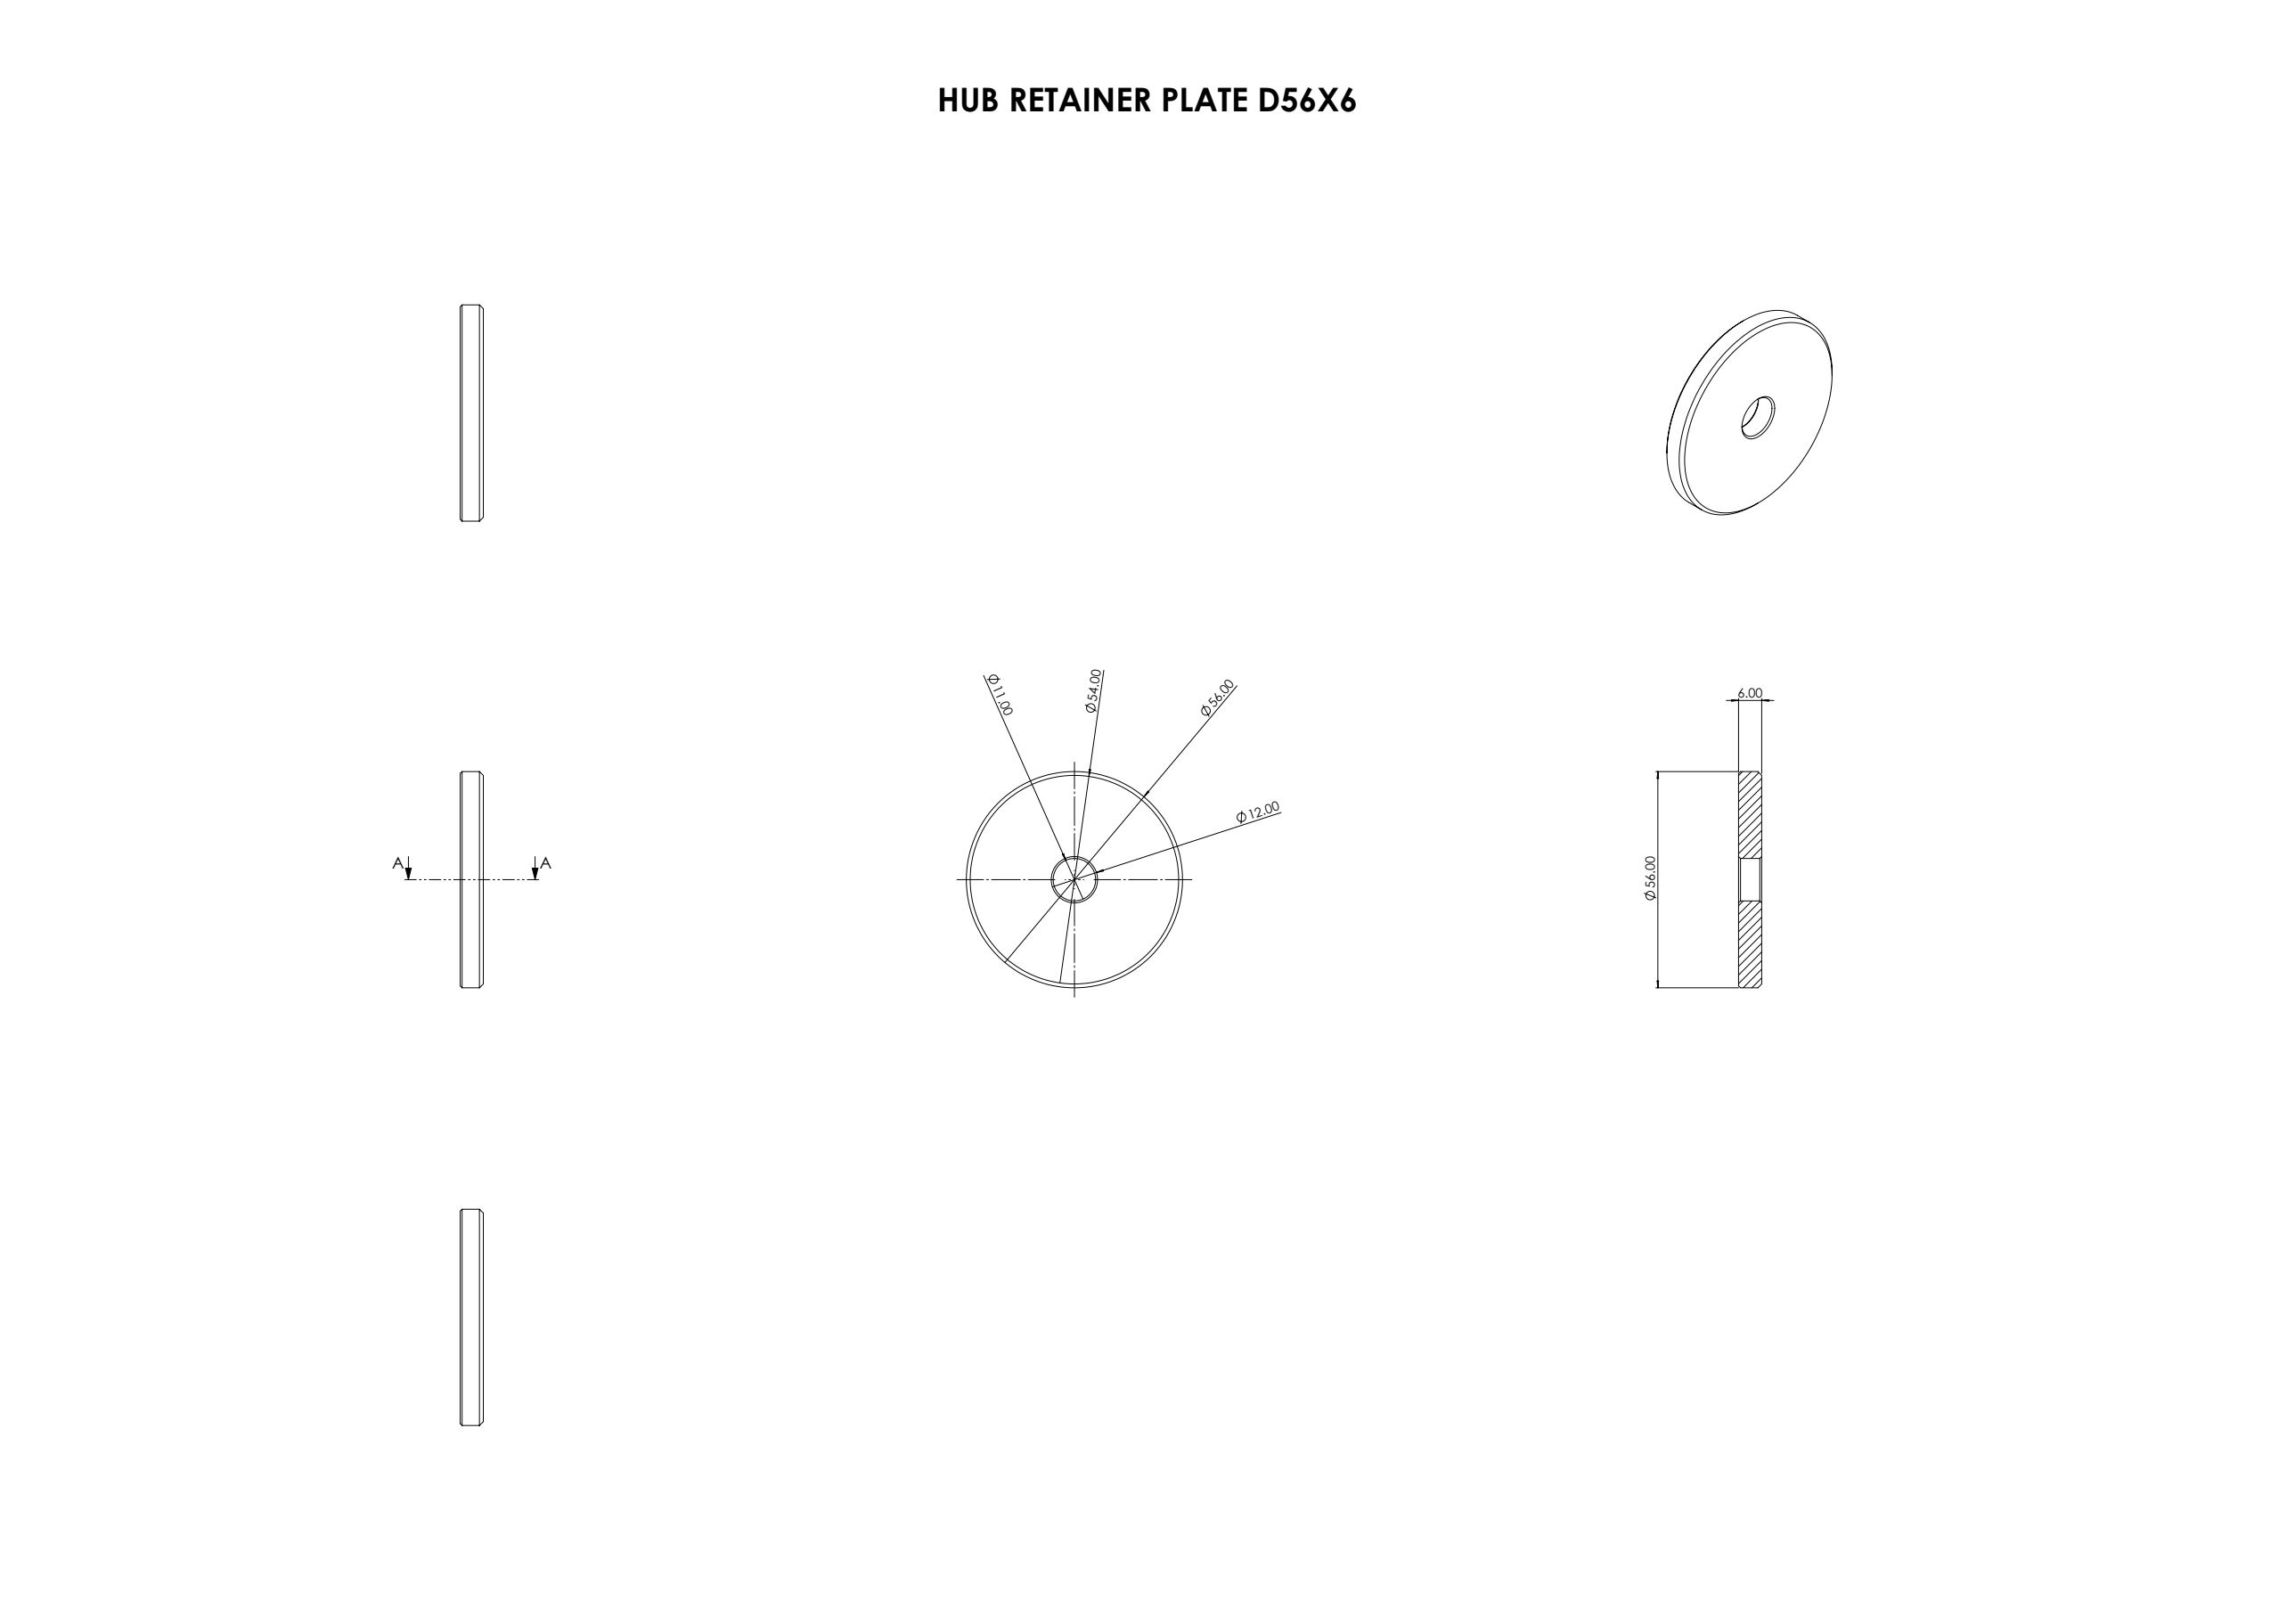
ISO-10303-21;
HEADER;
/* Generated by software containing ST-Developer
 * from STEP Tools, Inc. (www.steptools.com) 
 */

FILE_DESCRIPTION(
/* description */ (''),
/* implementation_level */ '2;1');

FILE_NAME(
/* name */ '05_Hub_Retainer_Plate_D56x6.step',
/* time_stamp */ '2026-10-11T08:27:52-07:00',
/* author */ (''),
/* organization */ (''),
/* preprocessor_version */ 'ST-DEVELOPER v20.2',
/* originating_system */ 'Autodesk Translation Framework v15.15.0.0',
/* authorisation */ '');

FILE_SCHEMA (('AUTOMOTIVE_DESIGN { 1 0 10303 214 3 1 1 }'));
ENDSEC;

DATA;
#10=MECHANICAL_DESIGN_GEOMETRIC_PRESENTATION_REPRESENTATION('',(#923),#94301);
#895=SHAPE_REPRESENTATION_RELATIONSHIP('SRR','None',#94375,#909);
#909=ADVANCED_BREP_SHAPE_REPRESENTATION('',(#937),#94291);
#923=STYLED_ITEM('',(#94574),#937);
#937=MANIFOLD_SOLID_BREP('Body1',#51022);
#1028=FACE_BOUND('',#18160,.T.);
#1029=FACE_BOUND('',#18165,.T.);
#1155=CYLINDRICAL_SURFACE('',#54475,5.5);
#1156=CYLINDRICAL_SURFACE('',#54484,28.);
#5973=LINE('',#84055,#10501);
#5974=LINE('',#84059,#10502);
#5975=LINE('',#84067,#10503);
#5976=LINE('',#84071,#10504);
#5977=LINE('',#84075,#10505);
#5978=LINE('',#84080,#10506);
#10501=VECTOR('',#65761,5.5);
#10502=VECTOR('',#65766,5.75);
#10503=VECTOR('',#65777,27.75);
#10504=VECTOR('',#65782,28.);
#10505=VECTOR('',#65787,27.5);
#10506=VECTOR('',#65794,5.75);
#12901=PLANE('',#54480);
#12902=PLANE('',#54488);
#15406=FACE_OUTER_BOUND('',#18157,.T.);
#15407=FACE_OUTER_BOUND('',#18158,.T.);
#15408=FACE_OUTER_BOUND('',#18159,.T.);
#15409=FACE_OUTER_BOUND('',#18161,.T.);
#15410=FACE_OUTER_BOUND('',#18162,.T.);
#15411=FACE_OUTER_BOUND('',#18163,.T.);
#15412=FACE_OUTER_BOUND('',#18164,.T.);
#15413=FACE_OUTER_BOUND('',#18166,.T.);
#18157=EDGE_LOOP('',(#45475,#45476,#45477,#45478));
#18158=EDGE_LOOP('',(#45479,#45480,#45481,#45482));
#18159=EDGE_LOOP('',(#45483));
#18160=EDGE_LOOP('',(#45484));
#18161=EDGE_LOOP('',(#45485,#45486,#45487,#45488));
#18162=EDGE_LOOP('',(#45489,#45490,#45491,#45492));
#18163=EDGE_LOOP('',(#45493,#45494,#45495,#45496));
#18164=EDGE_LOOP('',(#45497));
#18165=EDGE_LOOP('',(#45498));
#18166=EDGE_LOOP('',(#45499,#45500,#45501,#45502));
#20001=CIRCLE('',#54476,5.5);
#20002=CIRCLE('',#54477,5.5);
#20003=CIRCLE('',#54479,6.);
#20004=CIRCLE('',#54481,27.5);
#20005=CIRCLE('',#54483,28.);
#20006=CIRCLE('',#54485,28.);
#20007=CIRCLE('',#54487,27.);
#20008=CIRCLE('',#54489,6.);
#24498=VERTEX_POINT('',#84052);
#24499=VERTEX_POINT('',#84054);
#24500=VERTEX_POINT('',#84058);
#24501=VERTEX_POINT('',#84062);
#24502=VERTEX_POINT('',#84065);
#24503=VERTEX_POINT('',#84069);
#24504=VERTEX_POINT('',#84073);
#24505=VERTEX_POINT('',#84077);
#31599=EDGE_CURVE('',#24498,#24498,#20001,.T.);
#31600=EDGE_CURVE('',#24498,#24499,#5973,.T.);
#31601=EDGE_CURVE('',#24499,#24499,#20002,.T.);
#31602=EDGE_CURVE('',#24499,#24500,#5974,.T.);
#31603=EDGE_CURVE('',#24500,#24500,#20003,.T.);
#31604=EDGE_CURVE('',#24501,#24501,#20004,.T.);
#31605=EDGE_CURVE('',#24502,#24502,#20005,.T.);
#31606=EDGE_CURVE('',#24502,#24501,#5975,.T.);
#31607=EDGE_CURVE('',#24503,#24503,#20006,.T.);
#31608=EDGE_CURVE('',#24503,#24502,#5976,.T.);
#31609=EDGE_CURVE('',#24504,#24504,#20007,.T.);
#31610=EDGE_CURVE('',#24504,#24503,#5977,.T.);
#31611=EDGE_CURVE('',#24505,#24505,#20008,.T.);
#31612=EDGE_CURVE('',#24505,#24498,#5978,.T.);
#45475=ORIENTED_EDGE('',*,*,#31599,.T.);
#45476=ORIENTED_EDGE('',*,*,#31600,.T.);
#45477=ORIENTED_EDGE('',*,*,#31601,.F.);
#45478=ORIENTED_EDGE('',*,*,#31600,.F.);
#45479=ORIENTED_EDGE('',*,*,#31601,.T.);
#45480=ORIENTED_EDGE('',*,*,#31602,.T.);
#45481=ORIENTED_EDGE('',*,*,#31603,.F.);
#45482=ORIENTED_EDGE('',*,*,#31602,.F.);
#45483=ORIENTED_EDGE('',*,*,#31604,.F.);
#45484=ORIENTED_EDGE('',*,*,#31603,.T.);
#45485=ORIENTED_EDGE('',*,*,#31605,.F.);
#45486=ORIENTED_EDGE('',*,*,#31606,.T.);
#45487=ORIENTED_EDGE('',*,*,#31604,.T.);
#45488=ORIENTED_EDGE('',*,*,#31606,.F.);
#45489=ORIENTED_EDGE('',*,*,#31607,.F.);
#45490=ORIENTED_EDGE('',*,*,#31608,.T.);
#45491=ORIENTED_EDGE('',*,*,#31605,.T.);
#45492=ORIENTED_EDGE('',*,*,#31608,.F.);
#45493=ORIENTED_EDGE('',*,*,#31609,.F.);
#45494=ORIENTED_EDGE('',*,*,#31610,.T.);
#45495=ORIENTED_EDGE('',*,*,#31607,.T.);
#45496=ORIENTED_EDGE('',*,*,#31610,.F.);
#45497=ORIENTED_EDGE('',*,*,#31609,.T.);
#45498=ORIENTED_EDGE('',*,*,#31611,.F.);
#45499=ORIENTED_EDGE('',*,*,#31611,.T.);
#45500=ORIENTED_EDGE('',*,*,#31612,.T.);
#45501=ORIENTED_EDGE('',*,*,#31599,.F.);
#45502=ORIENTED_EDGE('',*,*,#31612,.F.);
#48302=CONICAL_SURFACE('',#54478,5.75,0.785398163397448);
#48303=CONICAL_SURFACE('',#54482,27.75,0.785398163397447);
#48304=CONICAL_SURFACE('',#54486,27.5,0.785398163397447);
#48305=CONICAL_SURFACE('',#54490,5.75,0.785398163397448);
#50493=ADVANCED_FACE('',(#15406),#1155,.F.);
#50494=ADVANCED_FACE('',(#15407),#48302,.F.);
#50495=ADVANCED_FACE('',(#15408,#1028),#12901,.T.);
#50496=ADVANCED_FACE('',(#15409),#48303,.T.);
#50497=ADVANCED_FACE('',(#15410),#1156,.T.);
#50498=ADVANCED_FACE('',(#15411),#48304,.T.);
#50499=ADVANCED_FACE('',(#15412,#1029),#12902,.T.);
#50500=ADVANCED_FACE('',(#15413),#48305,.F.);
#51022=CLOSED_SHELL('',(#50493,#50494,#50495,#50496,#50497,#50498,#50499,
#50500));
#54474=AXIS2_PLACEMENT_3D('',#84050,#65755,#65756);
#54475=AXIS2_PLACEMENT_3D('',#84051,#65757,#65758);
#54476=AXIS2_PLACEMENT_3D('',#84053,#65759,#65760);
#54477=AXIS2_PLACEMENT_3D('',#84056,#65762,#65763);
#54478=AXIS2_PLACEMENT_3D('',#84057,#65764,#65765);
#54479=AXIS2_PLACEMENT_3D('',#84060,#65767,#65768);
#54480=AXIS2_PLACEMENT_3D('',#84061,#65769,#65770);
#54481=AXIS2_PLACEMENT_3D('',#84063,#65771,#65772);
#54482=AXIS2_PLACEMENT_3D('',#84064,#65773,#65774);
#54483=AXIS2_PLACEMENT_3D('',#84066,#65775,#65776);
#54484=AXIS2_PLACEMENT_3D('',#84068,#65778,#65779);
#54485=AXIS2_PLACEMENT_3D('',#84070,#65780,#65781);
#54486=AXIS2_PLACEMENT_3D('',#84072,#65783,#65784);
#54487=AXIS2_PLACEMENT_3D('',#84074,#65785,#65786);
#54488=AXIS2_PLACEMENT_3D('',#84076,#65788,#65789);
#54489=AXIS2_PLACEMENT_3D('',#84078,#65790,#65791);
#54490=AXIS2_PLACEMENT_3D('',#84079,#65792,#65793);
#65755=DIRECTION('axis',(0.,0.,1.));
#65756=DIRECTION('refdir',(1.,0.,0.));
#65757=DIRECTION('center_axis',(1.,0.,0.));
#65758=DIRECTION('ref_axis',(0.,1.,0.));
#65759=DIRECTION('center_axis',(1.,0.,0.));
#65760=DIRECTION('ref_axis',(0.,0.,-1.));
#65761=DIRECTION('',(-1.,0.,0.));
#65762=DIRECTION('center_axis',(1.,0.,0.));
#65763=DIRECTION('ref_axis',(0.,0.,-1.));
#65764=DIRECTION('center_axis',(-1.,0.,0.));
#65765=DIRECTION('ref_axis',(0.,1.,0.));
#65766=DIRECTION('',(-0.707106781186548,-0.707106781186547,-8.65956056235493E-17));
#65767=DIRECTION('center_axis',(1.,0.,0.));
#65768=DIRECTION('ref_axis',(0.,0.,-1.));
#65769=DIRECTION('center_axis',(-1.,0.,0.));
#65770=DIRECTION('ref_axis',(0.,0.,1.));
#65771=DIRECTION('center_axis',(1.,0.,0.));
#65772=DIRECTION('ref_axis',(0.,0.,-1.));
#65773=DIRECTION('center_axis',(1.,0.,0.));
#65774=DIRECTION('ref_axis',(0.,1.,0.));
#65775=DIRECTION('center_axis',(1.,0.,0.));
#65776=DIRECTION('ref_axis',(0.,0.,-1.));
#65777=DIRECTION('',(-0.707106781186549,0.707106781186546,8.65956056235492E-17));
#65778=DIRECTION('center_axis',(1.,0.,0.));
#65779=DIRECTION('ref_axis',(0.,1.,0.));
#65780=DIRECTION('center_axis',(1.,0.,0.));
#65781=DIRECTION('ref_axis',(0.,0.,-1.));
#65782=DIRECTION('',(-1.,0.,0.));
#65783=DIRECTION('center_axis',(-1.,0.,0.));
#65784=DIRECTION('ref_axis',(0.,1.,0.));
#65785=DIRECTION('center_axis',(1.,0.,0.));
#65786=DIRECTION('ref_axis',(0.,0.,-1.));
#65787=DIRECTION('',(-0.707106781186549,-0.707106781186546,-8.65956056235492E-17));
#65788=DIRECTION('center_axis',(1.,0.,0.));
#65789=DIRECTION('ref_axis',(0.,0.,-1.));
#65790=DIRECTION('center_axis',(1.,0.,0.));
#65791=DIRECTION('ref_axis',(0.,0.,-1.));
#65792=DIRECTION('center_axis',(1.,0.,0.));
#65793=DIRECTION('ref_axis',(0.,1.,0.));
#65794=DIRECTION('',(-0.707106781186548,0.707106781186548,8.65956056235493E-17));
#84050=CARTESIAN_POINT('',(0.,0.,0.));
#84051=CARTESIAN_POINT('Origin',(3.,0.,0.));
#84052=CARTESIAN_POINT('',(5.5,-5.5,-6.73555739531044E-16));
#84053=CARTESIAN_POINT('Origin',(5.5,0.,0.));
#84054=CARTESIAN_POINT('',(0.5,-5.5,-6.73555739531044E-16));
#84055=CARTESIAN_POINT('',(3.,-5.5,-6.73555739531044E-16));
#84056=CARTESIAN_POINT('Origin',(0.5,0.,0.));
#84057=CARTESIAN_POINT('Origin',(0.25,0.,0.));
#84058=CARTESIAN_POINT('',(-2.42861286636753E-16,-6.,-7.34788079488412E-16));
#84059=CARTESIAN_POINT('',(0.25,-5.75,-7.04171909509728E-16));
#84060=CARTESIAN_POINT('Origin',(0.,0.,0.));
#84061=CARTESIAN_POINT('Origin',(0.,27.5,0.));
#84062=CARTESIAN_POINT('',(-7.63278329429795E-16,-27.5,-3.36777869765522E-15));
#84063=CARTESIAN_POINT('Origin',(0.,0.,0.));
#84064=CARTESIAN_POINT('Origin',(0.25,0.,0.));
#84065=CARTESIAN_POINT('',(0.500000000000002,-28.,-3.42901103761259E-15));
#84066=CARTESIAN_POINT('Origin',(0.5,0.,0.));
#84067=CARTESIAN_POINT('',(0.25,-27.75,-3.39839486763391E-15));
#84068=CARTESIAN_POINT('Origin',(2.75,0.,0.));
#84069=CARTESIAN_POINT('',(5.,-28.,-3.42901103761259E-15));
#84070=CARTESIAN_POINT('Origin',(5.,0.,0.));
#84071=CARTESIAN_POINT('',(2.75,-28.,-3.42901103761259E-15));
#84072=CARTESIAN_POINT('Origin',(5.5,0.,0.));
#84073=CARTESIAN_POINT('',(6.,-27.,-3.30654635769785E-15));
#84074=CARTESIAN_POINT('Origin',(6.,0.,0.));
#84075=CARTESIAN_POINT('',(5.5,-27.5,-3.36777869765522E-15));
#84076=CARTESIAN_POINT('Origin',(6.,6.,0.));
#84077=CARTESIAN_POINT('',(6.,-6.,-7.34788079488412E-16));
#84078=CARTESIAN_POINT('Origin',(6.,0.,0.));
#84079=CARTESIAN_POINT('Origin',(5.75,0.,0.));
#84080=CARTESIAN_POINT('',(5.75,-5.75,-7.04171909509728E-16));
#94275=UNCERTAINTY_MEASURE_WITH_UNIT(LENGTH_MEASURE(0.01),#94302,
'DISTANCE_ACCURACY_VALUE',
'Maximum model space distance between geometric entities at asserted c
onnectivities');
#94285=UNCERTAINTY_MEASURE_WITH_UNIT(LENGTH_MEASURE(0.01),#94302,
'DISTANCE_ACCURACY_VALUE',
'Maximum model space distance between geometric entities at asserted c
onnectivities');
#94291=(
GEOMETRIC_REPRESENTATION_CONTEXT(3)
GLOBAL_UNCERTAINTY_ASSIGNED_CONTEXT((#94275))
GLOBAL_UNIT_ASSIGNED_CONTEXT((#94302,#94304,#94305))
REPRESENTATION_CONTEXT('','3D')
);
#94301=(
GEOMETRIC_REPRESENTATION_CONTEXT(3)
GLOBAL_UNCERTAINTY_ASSIGNED_CONTEXT((#94285))
GLOBAL_UNIT_ASSIGNED_CONTEXT((#94302,#94304,#94305))
REPRESENTATION_CONTEXT('','3D')
);
#94302=(
LENGTH_UNIT()
NAMED_UNIT(*)
SI_UNIT(.MILLI.,.METRE.)
);
#94304=(
NAMED_UNIT(*)
PLANE_ANGLE_UNIT()
SI_UNIT($,.RADIAN.)
);
#94305=(
NAMED_UNIT(*)
SI_UNIT($,.STERADIAN.)
SOLID_ANGLE_UNIT()
);
#94311=SHAPE_DEFINITION_REPRESENTATION(#94326,#94375);
#94326=PRODUCT_DEFINITION_SHAPE('',$,#94391);
#94375=SHAPE_REPRESENTATION('',(#54474),#94291);
#94385=PRODUCT_DEFINITION_CONTEXT('part definition',#94432,'design');
#94391=PRODUCT_DEFINITION('2026-10-11-08-26-38-347',
'05_Hub_Retainer_Plate_D56x6',#94406,#94385);
#94406=PRODUCT_DEFINITION_FORMATION('',$,#94439);
#94432=APPLICATION_CONTEXT(
'Core Data for Automotive Mechanical Design Process');
#94433=PRODUCT_CONTEXT('part definition',#94432,'mechanical');
#94439=PRODUCT('2026-10-11-08-26-38-347','05_Hub_Retainer_Plate_D56x6',
$,(#94433));
#94568=COLOUR_RGB('Sky Blue',0.24,0.69,0.87);
#94569=FILL_AREA_STYLE_COLOUR('',#94568);
#94570=FILL_AREA_STYLE('',(#94569));
#94571=SURFACE_STYLE_FILL_AREA(#94570);
#94572=SURFACE_SIDE_STYLE('',(#94571));
#94573=SURFACE_STYLE_USAGE(.BOTH.,#94572);
#94574=PRESENTATION_STYLE_ASSIGNMENT((#94573));
ENDSEC;
END-ISO-10303-21;
